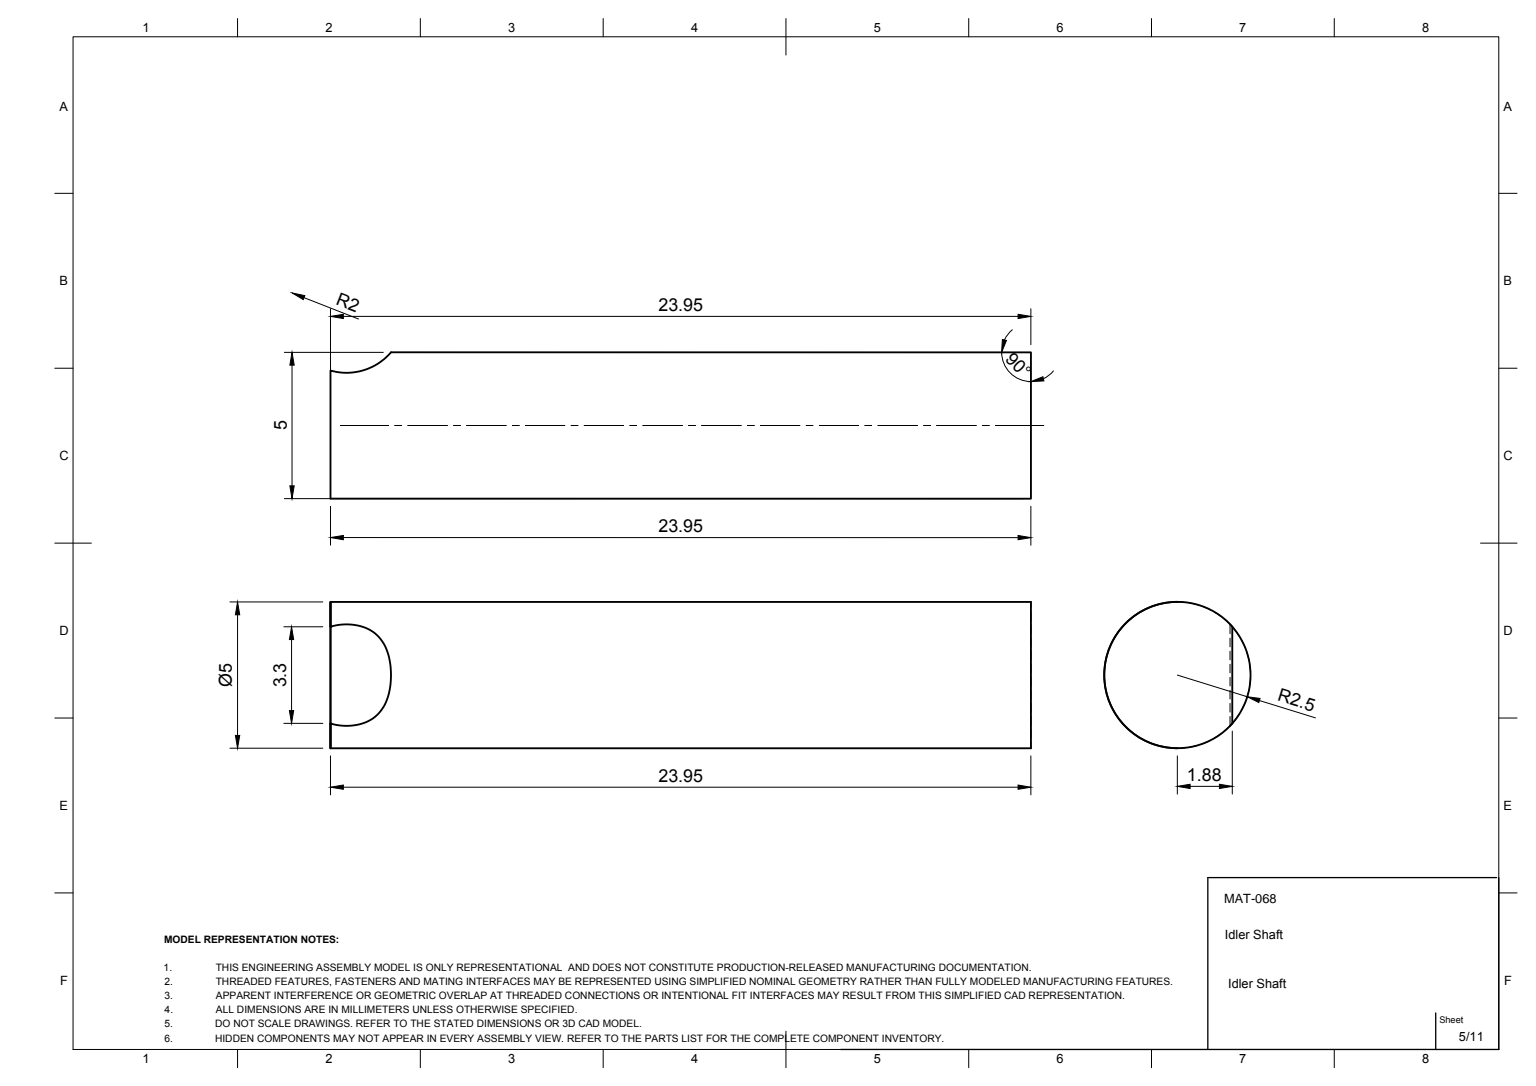
ISO-10303-21;
HEADER;
/* Generated by software containing ST-Developer
 * from STEP Tools, Inc. (www.steptools.com) 
 */

FILE_DESCRIPTION(
/* description */ ('CAx-IF Rec.Pracs.---Representation and Presentation of Product Manufa
cturing Information (PMI)---4.0---2014-10-13'),
/* implementation_level */ '2;1');

FILE_NAME(
/* name */ 'Idler Shaft.step',
/* time_stamp */ '2026-10-24T16:53:48-07:00',
/* author */ (''),
/* organization */ (''),
/* preprocessor_version */ 'ST-DEVELOPER v20.2',
/* originating_system */ 'Autodesk Translation Framework v15.17.0.0',
/* authorisation */ '');

FILE_SCHEMA (('AP242_MANAGED_MODEL_BASED_3D_ENGINEERING_MIM_LF { 1 0 10303 442 2 1 4 }'));
ENDSEC;

DATA;
#10=MECHANICAL_DESIGN_GEOMETRIC_PRESENTATION_REPRESENTATION('',(#3492),#107910);
#1141=B_SPLINE_CURVE_WITH_KNOTS('',3,(#63387,#63388,#63389,#63390,#63391,
#63392,#63393,#63394,#63395,#63396,#63397,#63398,#63399,#63400,#63401,#63402,
#63403,#63404,#63405,#63406,#63407,#63408,#63409,#63410,#63411,#63412,#63413),
 .UNSPECIFIED.,.F.,.F.,(4,3,2,2,2,2,2,2,2,2,2,2,4),(-0.0542367397696986,
0.,0.0558778999014289,0.111755799802858,0.16455192751495,0.212643516719156,
0.260735105923363,0.308826695127569,0.356918284331776,0.409714412043867,
0.465592311945296,0.521470211846725,0.575706951616422),.UNSPECIFIED.);
#3472=SHAPE_REPRESENTATION_RELATIONSHIP('SRR','None',#107950,#3482);
#3482=ADVANCED_BREP_SHAPE_REPRESENTATION('',(#3502),#107903);
#3492=STYLED_ITEM('',(#108009),#3502);
#3502=MANIFOLD_SOLID_BREP('Body1',#45540);
#3548=PLANE('',#45685);
#3549=PLANE('',#45686);
#3769=FACE_OUTER_BOUND('',#6695,.T.);
#3770=FACE_OUTER_BOUND('',#6696,.T.);
#3771=FACE_OUTER_BOUND('',#6697,.T.);
#3772=FACE_OUTER_BOUND('',#6698,.T.);
#6695=EDGE_LOOP('',(#28152,#28153,#28154,#28155,#28156,#28157));
#6696=EDGE_LOOP('',(#28158,#28159,#28160));
#6697=EDGE_LOOP('',(#28161));
#6698=EDGE_LOOP('',(#28162,#28163));
#9642=LINE('',#63383,#11626);
#9643=LINE('',#63416,#11627);
#11626=VECTOR('',#50429,0.0025);
#11627=VECTOR('',#50436,1.);
#13615=CIRCLE('',#45682,0.00250000000001001);
#13616=CIRCLE('',#45683,0.00250000000001001);
#13617=CIRCLE('',#45684,0.00250000000001001);
#17189=VERTEX_POINT('',#63380);
#17190=VERTEX_POINT('',#63382);
#17191=VERTEX_POINT('',#63384);
#17192=VERTEX_POINT('',#63386);
#21218=EDGE_CURVE('',#17189,#17189,#13615,.T.);
#21219=EDGE_CURVE('',#17189,#17190,#9642,.T.);
#21220=EDGE_CURVE('',#17190,#17191,#13616,.T.);
#21221=EDGE_CURVE('',#17192,#17191,#1141,.F.);
#21222=EDGE_CURVE('',#17192,#17190,#13617,.T.);
#21223=EDGE_CURVE('',#17192,#17191,#9643,.T.);
#28152=ORIENTED_EDGE('',*,*,#21218,.F.);
#28153=ORIENTED_EDGE('',*,*,#21219,.T.);
#28154=ORIENTED_EDGE('',*,*,#21220,.T.);
#28155=ORIENTED_EDGE('',*,*,#21221,.F.);
#28156=ORIENTED_EDGE('',*,*,#21222,.T.);
#28157=ORIENTED_EDGE('',*,*,#21219,.F.);
#28158=ORIENTED_EDGE('',*,*,#21222,.F.);
#28159=ORIENTED_EDGE('',*,*,#21223,.T.);
#28160=ORIENTED_EDGE('',*,*,#21220,.F.);
#28161=ORIENTED_EDGE('',*,*,#21218,.T.);
#28162=ORIENTED_EDGE('',*,*,#21221,.T.);
#28163=ORIENTED_EDGE('',*,*,#21223,.F.);
#41963=CYLINDRICAL_SURFACE('',#45681,0.0025);
#41964=CYLINDRICAL_SURFACE('',#45687,0.002);
#42624=ADVANCED_FACE('',(#3769),#41963,.T.);
#42625=ADVANCED_FACE('',(#3770),#3548,.F.);
#42626=ADVANCED_FACE('',(#3771),#3549,.T.);
#42627=ADVANCED_FACE('',(#3772),#41964,.F.);
#45540=CLOSED_SHELL('',(#42624,#42625,#42626,#42627));
#45680=AXIS2_PLACEMENT_3D('',#63378,#50423,#50424);
#45681=AXIS2_PLACEMENT_3D('',#63379,#50425,#50426);
#45682=AXIS2_PLACEMENT_3D('',#63381,#50427,#50428);
#45683=AXIS2_PLACEMENT_3D('',#63385,#50430,#50431);
#45684=AXIS2_PLACEMENT_3D('',#63414,#50432,#50433);
#45685=AXIS2_PLACEMENT_3D('',#63415,#50434,#50435);
#45686=AXIS2_PLACEMENT_3D('',#63417,#50437,#50438);
#45687=AXIS2_PLACEMENT_3D('',#63418,#50439,#50440);
#50423=DIRECTION('axis',(0.,0.,1.));
#50424=DIRECTION('refdir',(1.,0.,0.));
#50425=DIRECTION('center_axis',(0.,0.,-1.));
#50426=DIRECTION('ref_axis',(-1.,0.,0.));
#50427=DIRECTION('center_axis',(0.,0.,-1.));
#50428=DIRECTION('ref_axis',(-1.,0.,0.));
#50429=DIRECTION('',(0.,0.,1.));
#50430=DIRECTION('center_axis',(0.,0.,-1.));
#50431=DIRECTION('ref_axis',(-1.,0.,0.));
#50432=DIRECTION('center_axis',(0.,0.,-1.));
#50433=DIRECTION('ref_axis',(-1.,0.,0.));
#50434=DIRECTION('center_axis',(0.,0.,-1.));
#50435=DIRECTION('ref_axis',(0.,-1.,0.));
#50436=DIRECTION('',(1.,0.,0.));
#50437=DIRECTION('center_axis',(0.,0.,-1.));
#50438=DIRECTION('ref_axis',(0.,-1.,0.));
#50439=DIRECTION('center_axis',(1.,0.,0.));
#50440=DIRECTION('ref_axis',(0.,0.,-1.));
#63378=CARTESIAN_POINT('',(0.,0.,0.));
#63379=CARTESIAN_POINT('Origin',(-0.00312621780689159,0.00227581852803817,
0.0795478161976335));
#63380=CARTESIAN_POINT('',(-0.00062621780689159,0.00227581852803817,0.05560000000001));
#63381=CARTESIAN_POINT('Origin',(-0.0031262178069016,0.00227581852804816,
0.05560000000001));
#63382=CARTESIAN_POINT('',(-0.00062621780689159,0.00227581852803817,0.0795478161976436));
#63383=CARTESIAN_POINT('',(-0.00062621780689159,0.00227581852803817,0.0795478161976335));
#63384=CARTESIAN_POINT('',(-0.00147431229815866,0.000399330267958239,0.0795478161976335));
#63385=CARTESIAN_POINT('Origin',(-0.0031262178069016,0.00227581852804816,
0.0795478161976436));
#63386=CARTESIAN_POINT('',(-0.00477812331562454,0.000399330267958239,0.0795478161976335));
#63387=CARTESIAN_POINT('Ctrl Pts',(-0.00147431229815864,0.000399330267958261,
0.0795478161976335));
#63388=CARTESIAN_POINT('Ctrl Pts',(-0.00141756753743531,0.000449283675514679,
0.0793724180142668));
#63389=CARTESIAN_POINT('Ctrl Pts',(-0.00139128264960183,0.00047581852803818,
0.0791807891325657));
#63390=CARTESIAN_POINT('Ctrl Pts',(-0.00139128264960183,0.00047581852803818,
0.079));
#63391=CARTESIAN_POINT('Ctrl Pts',(-0.00139128264960183,0.00047581852803818,
0.0788137403336619));
#63392=CARTESIAN_POINT('Ctrl Pts',(-0.00141923484858738,0.000447531815482377,
0.0786160265927576));
#63393=CARTESIAN_POINT('Ctrl Pts',(-0.00153985493559125,0.000341941867351019,
0.0782565826026003));
#63394=CARTESIAN_POINT('Ctrl Pts',(-0.00163385434425655,0.000265418371407152,
0.0780950718110287));
#63395=CARTESIAN_POINT('Ctrl Pts',(-0.00185670743308821,0.000118232327801343,
0.0778503362730228));
#63396=CARTESIAN_POINT('Ctrl Pts',(-0.00201374560920302,3.11585522271903E-5,
0.0777391784281712));
#63397=CARTESIAN_POINT('Ctrl Pts',(-0.00229857646949163,-8.77930433005222E-5,
0.0776057075686815));
#63398=CARTESIAN_POINT('Ctrl Pts',(-0.00245822273383093,-0.000139297746093857,
0.0775563101781988));
#63399=CARTESIAN_POINT('Ctrl Pts',(-0.00279192215600469,-0.000207576533398147,
0.0774937815188223));
#63400=CARTESIAN_POINT('Ctrl Pts',(-0.00296591250954424,-0.00022418147196183,
0.0774801315846429));
#63401=CARTESIAN_POINT('Ctrl Pts',(-0.00328652310423895,-0.00022418147196183,
0.0774801315846429));
#63402=CARTESIAN_POINT('Ctrl Pts',(-0.0034605134577785,-0.000207576533398146,
0.0774937815188223));
#63403=CARTESIAN_POINT('Ctrl Pts',(-0.00379421287995226,-0.000139297746093855,
0.0775563101781988));
#63404=CARTESIAN_POINT('Ctrl Pts',(-0.00395385914429156,-8.77930433005201E-5,
0.0776057075686815));
#63405=CARTESIAN_POINT('Ctrl Pts',(-0.00423869000458017,3.11585522271924E-5,
0.0777391784281712));
#63406=CARTESIAN_POINT('Ctrl Pts',(-0.00439572818069498,0.000118232327801344,
0.0778503362730228));
#63407=CARTESIAN_POINT('Ctrl Pts',(-0.00461858126952663,0.000265418371407153,
0.0780950718110287));
#63408=CARTESIAN_POINT('Ctrl Pts',(-0.00471258067819193,0.000341941867351019,
0.0782565826026003));
#63409=CARTESIAN_POINT('Ctrl Pts',(-0.0048332007651958,0.000447531815482377,
0.0786160265927576));
#63410=CARTESIAN_POINT('Ctrl Pts',(-0.00486115296418135,0.00047581852803818,
0.0788137403336619));
#63411=CARTESIAN_POINT('Ctrl Pts',(-0.00486115296418135,0.00047581852803818,
0.0791807891325657));
#63412=CARTESIAN_POINT('Ctrl Pts',(-0.00483486807634788,0.000449283675514682,
0.0793724180142668));
#63413=CARTESIAN_POINT('Ctrl Pts',(-0.00477812331562455,0.000399330267958265,
0.0795478161976335));
#63414=CARTESIAN_POINT('Origin',(-0.0031262178069016,0.00227581852804816,
0.0795478161976436));
#63415=CARTESIAN_POINT('Origin',(-0.00312621780689159,0.00227581852803817,
0.0795478161976335));
#63416=CARTESIAN_POINT('',(-0.0411262178069016,0.000399330267968239,0.0795478161976436));
#63417=CARTESIAN_POINT('Origin',(-0.00312621780689159,0.00227581852803817,
0.0556));
#63418=CARTESIAN_POINT('Origin',(-0.0411262178068916,-0.00152418147196182,
0.079));
#107891=UNCERTAINTY_MEASURE_WITH_UNIT(LENGTH_MEASURE(1.E-5),#107911,
'DISTANCE_ACCURACY_VALUE',
'Maximum model space distance between geometric entities at asserted c
onnectivities');
#107898=UNCERTAINTY_MEASURE_WITH_UNIT(LENGTH_MEASURE(1.E-5),#107911,
'DISTANCE_ACCURACY_VALUE',
'Maximum model space distance between geometric entities at asserted c
onnectivities');
#107903=(
GEOMETRIC_REPRESENTATION_CONTEXT(3)
GLOBAL_UNCERTAINTY_ASSIGNED_CONTEXT((#107891))
GLOBAL_UNIT_ASSIGNED_CONTEXT((#107911,#107912,#107913))
REPRESENTATION_CONTEXT('','3D')
);
#107910=(
GEOMETRIC_REPRESENTATION_CONTEXT(3)
GLOBAL_UNCERTAINTY_ASSIGNED_CONTEXT((#107898))
GLOBAL_UNIT_ASSIGNED_CONTEXT((#107911,#107912,#107913))
REPRESENTATION_CONTEXT('','3D')
);
#107911=(
LENGTH_UNIT()
NAMED_UNIT(*)
SI_UNIT($,.METRE.)
);
#107912=(
NAMED_UNIT(*)
PLANE_ANGLE_UNIT()
SI_UNIT($,.RADIAN.)
);
#107913=(
NAMED_UNIT(*)
SI_UNIT($,.STERADIAN.)
SOLID_ANGLE_UNIT()
);
#107918=SHAPE_DEFINITION_REPRESENTATION(#107929,#107950);
#107929=PRODUCT_DEFINITION_SHAPE('',$,#107962);
#107950=SHAPE_REPRESENTATION('',(#45680),#107903);
#107957=PRODUCT_DEFINITION_CONTEXT('part definition',#107992,'design');
#107962=PRODUCT_DEFINITION('Idler Shaft','Idler Shaft',#107973,#107957);
#107973=PRODUCT_DEFINITION_FORMATION('',$,#107998);
#107992=APPLICATION_CONTEXT('Managed model based 3d engineering');
#107993=PRODUCT_CONTEXT('part definition',#107992,'mechanical');
#107998=PRODUCT('Idler Shaft','Idler Shaft',
'LEGAL AND USAGE DISCLAIMER: this Data/Model is provided \X2\201C\X0\A
S IS\X2\201D\X0\ for informational and representational only. It is a 
geometric approximation and is NOT engineered, certified, or guarantee
d for dimensional accuracy, exact tolerances, or production-level prec
ision. Vendor disclaims all implied warranties including fitness for a
 particular purpose. DO NOT USE FOR DIRECT PHYSICAL MANUFACTURING, AUT
OMATED PRODUCTION, OR SAFETY-CRITICAL SYSTEMS without independent engi
neering verification and resolution of any design discrepancies.',(#107993));
#108009=PRESENTATION_STYLE_ASSIGNMENT((#108016));
#108016=SURFACE_STYLE_USAGE(.BOTH.,#108023);
#108023=SURFACE_SIDE_STYLE('',(#108030));
#108030=SURFACE_STYLE_FILL_AREA(#108037);
#108037=FILL_AREA_STYLE('Opaque(179,179,179)',(#108044));
#108044=FILL_AREA_STYLE_COLOUR('Opaque(179,179,179)',#108051);
#108051=COLOUR_RGB('Opaque(179,179,179)',0.701960784313725,0.701960784313725,
0.701960784313725);
ENDSEC;
END-ISO-10303-21;
